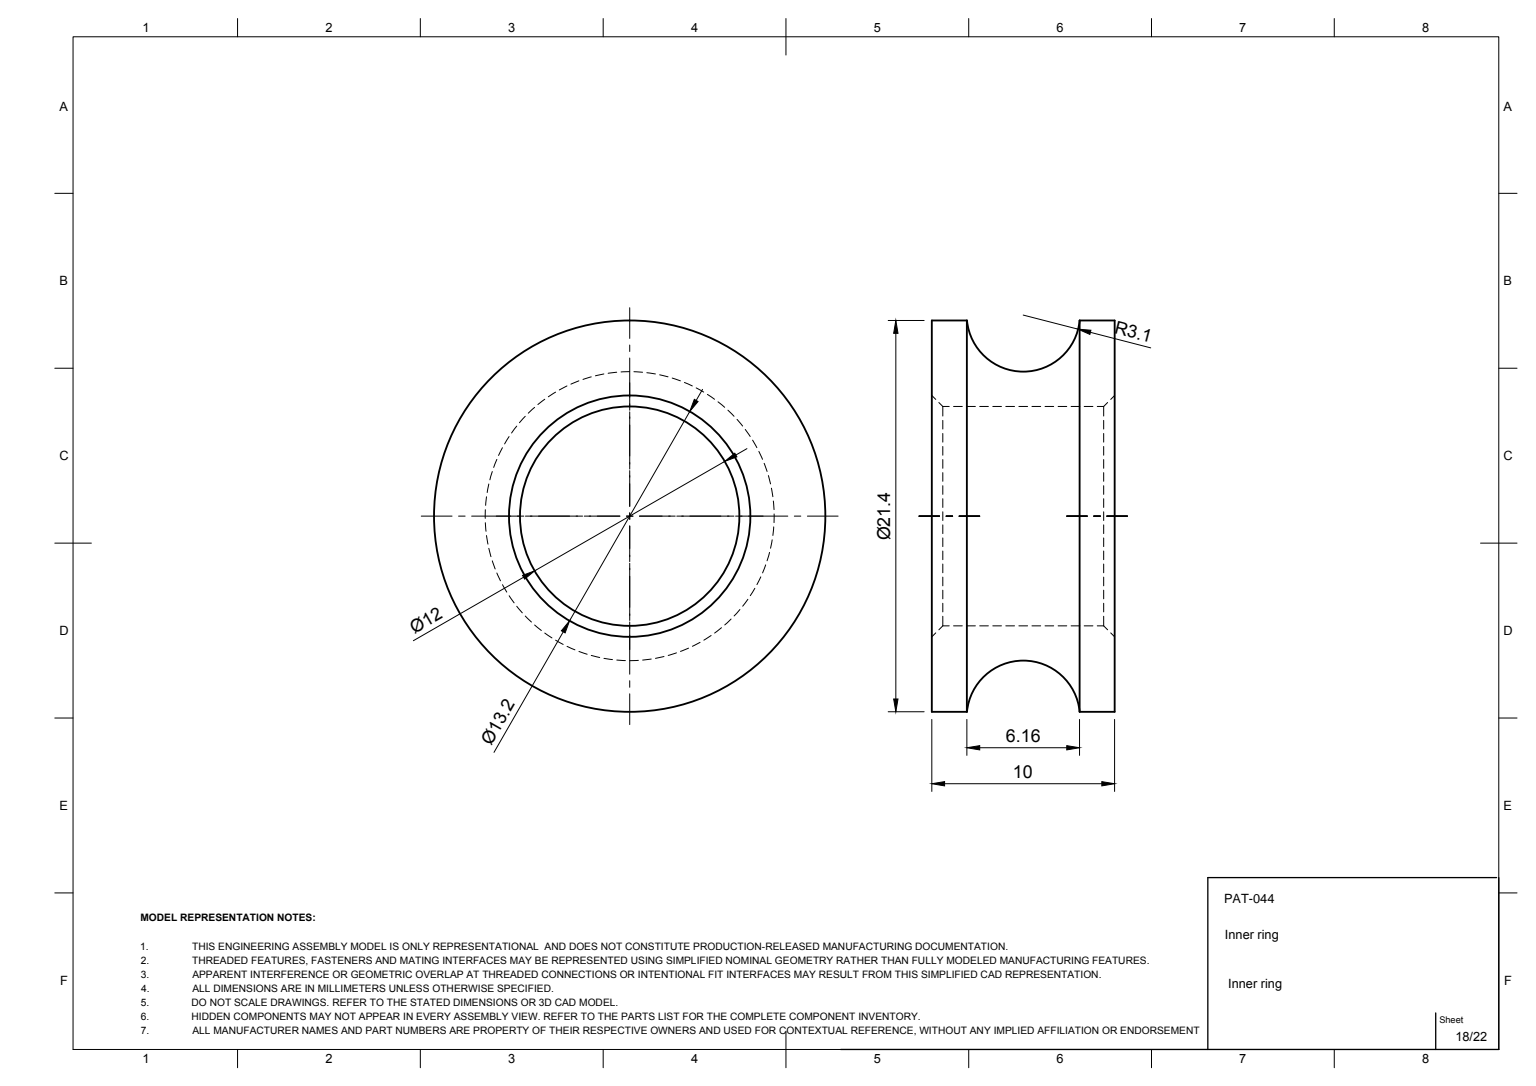
ISO-10303-21;
HEADER;
/* Generated by software containing ST-Developer
 * from STEP Tools, Inc. (www.steptools.com) 
 */

FILE_DESCRIPTION(
/* description */ ('Four-wheel beam trolley'),
/* implementation_level */ '2;1');

FILE_NAME(
/* name */ 'Inner ring.step',
/* time_stamp */ '2026-10-29T16:22:06-07:00',
/* author */ (''),
/* organization */ (''),
/* preprocessor_version */ 'ST-DEVELOPER v20.2',
/* originating_system */ 'Autodesk Translation Framework v15.17.0.0',
/* authorisation */ '');

FILE_SCHEMA (('AUTOMOTIVE_DESIGN { 1 0 10303 214 3 1 1 }'));
ENDSEC;

DATA;
#10=MECHANICAL_DESIGN_GEOMETRIC_PRESENTATION_REPRESENTATION('',(#289),#4777);
#39=TOROIDAL_SURFACE('',#2787,1.1,0.309556);
#238=CONICAL_SURFACE('',#2798,0.63,0.785398163397448);
#239=CONICAL_SURFACE('',#2805,0.63,0.785398163397448);
#255=SHAPE_REPRESENTATION_RELATIONSHIP('SRR','None',#4886,#272);
#272=ADVANCED_BREP_SHAPE_REPRESENTATION('',(#311),#4771);
#289=STYLED_ITEM('',(#5056),#311);
#311=MANIFOLD_SOLID_BREP('Body1',#2378);
#354=FACE_BOUND('',#719,.T.);
#355=FACE_BOUND('',#722,.T.);
#424=PLANE('',#2800);
#425=PLANE('',#2803);
#537=FACE_OUTER_BOUND('',#714,.T.);
#538=FACE_OUTER_BOUND('',#715,.T.);
#539=FACE_OUTER_BOUND('',#716,.T.);
#540=FACE_OUTER_BOUND('',#717,.T.);
#541=FACE_OUTER_BOUND('',#718,.T.);
#542=FACE_OUTER_BOUND('',#720,.T.);
#543=FACE_OUTER_BOUND('',#721,.T.);
#544=FACE_OUTER_BOUND('',#723,.T.);
#714=EDGE_LOOP('',(#1965,#1966,#1967,#1968,#1969,#1970));
#715=EDGE_LOOP('',(#1971,#1972,#1973,#1974,#1975));
#716=EDGE_LOOP('',(#1976,#1977,#1978,#1979));
#717=EDGE_LOOP('',(#1980,#1981,#1982,#1983));
#718=EDGE_LOOP('',(#1984));
#719=EDGE_LOOP('',(#1985));
#720=EDGE_LOOP('',(#1986,#1987,#1988,#1989,#1990));
#721=EDGE_LOOP('',(#1991));
#722=EDGE_LOOP('',(#1992));
#723=EDGE_LOOP('',(#1993,#1994,#1995,#1996));
#882=LINE('',#4197,#1005);
#883=LINE('',#4203,#1006);
#884=LINE('',#4207,#1007);
#885=LINE('',#4213,#1008);
#886=LINE('',#4218,#1009);
#1005=VECTOR('',#3467,1.070235);
#1006=VECTOR('',#3474,0.6);
#1007=VECTOR('',#3479,0.63);
#1008=VECTOR('',#3488,1.070235);
#1009=VECTOR('',#3495,0.63);
#1088=CIRCLE('',#2788,1.070235);
#1089=CIRCLE('',#2789,1.070235);
#1090=CIRCLE('',#2790,0.309556);
#1091=CIRCLE('',#2791,1.070235);
#1092=CIRCLE('',#2792,1.070235);
#1093=CIRCLE('',#2794,1.070235);
#1094=CIRCLE('',#2796,0.6);
#1095=CIRCLE('',#2797,0.6);
#1096=CIRCLE('',#2799,0.66);
#1097=CIRCLE('',#2802,1.070235);
#1098=CIRCLE('',#2804,0.66);
#1272=VERTEX_POINT('',#4186);
#1273=VERTEX_POINT('',#4187);
#1274=VERTEX_POINT('',#4190);
#1275=VERTEX_POINT('',#4192);
#1276=VERTEX_POINT('',#4196);
#1277=VERTEX_POINT('',#4200);
#1278=VERTEX_POINT('',#4202);
#1279=VERTEX_POINT('',#4206);
#1280=VERTEX_POINT('',#4211);
#1281=VERTEX_POINT('',#4215);
#1520=EDGE_CURVE('',#1272,#1273,#1088,.T.);
#1521=EDGE_CURVE('',#1273,#1272,#1089,.T.);
#1522=EDGE_CURVE('',#1273,#1274,#1090,.T.);
#1523=EDGE_CURVE('',#1275,#1274,#1091,.T.);
#1524=EDGE_CURVE('',#1274,#1275,#1092,.T.);
#1525=EDGE_CURVE('',#1275,#1276,#882,.T.);
#1526=EDGE_CURVE('',#1276,#1276,#1093,.T.);
#1527=EDGE_CURVE('',#1277,#1277,#1094,.T.);
#1528=EDGE_CURVE('',#1277,#1278,#883,.T.);
#1529=EDGE_CURVE('',#1278,#1278,#1095,.T.);
#1530=EDGE_CURVE('',#1278,#1279,#884,.T.);
#1531=EDGE_CURVE('',#1279,#1279,#1096,.T.);
#1532=EDGE_CURVE('',#1280,#1280,#1097,.T.);
#1533=EDGE_CURVE('',#1280,#1272,#885,.T.);
#1534=EDGE_CURVE('',#1281,#1281,#1098,.T.);
#1535=EDGE_CURVE('',#1281,#1277,#886,.T.);
#1965=ORIENTED_EDGE('',*,*,#1520,.F.);
#1966=ORIENTED_EDGE('',*,*,#1521,.F.);
#1967=ORIENTED_EDGE('',*,*,#1522,.T.);
#1968=ORIENTED_EDGE('',*,*,#1523,.F.);
#1969=ORIENTED_EDGE('',*,*,#1524,.F.);
#1970=ORIENTED_EDGE('',*,*,#1522,.F.);
#1971=ORIENTED_EDGE('',*,*,#1523,.T.);
#1972=ORIENTED_EDGE('',*,*,#1524,.T.);
#1973=ORIENTED_EDGE('',*,*,#1525,.T.);
#1974=ORIENTED_EDGE('',*,*,#1526,.T.);
#1975=ORIENTED_EDGE('',*,*,#1525,.F.);
#1976=ORIENTED_EDGE('',*,*,#1527,.T.);
#1977=ORIENTED_EDGE('',*,*,#1528,.T.);
#1978=ORIENTED_EDGE('',*,*,#1529,.F.);
#1979=ORIENTED_EDGE('',*,*,#1528,.F.);
#1980=ORIENTED_EDGE('',*,*,#1529,.T.);
#1981=ORIENTED_EDGE('',*,*,#1530,.T.);
#1982=ORIENTED_EDGE('',*,*,#1531,.F.);
#1983=ORIENTED_EDGE('',*,*,#1530,.F.);
#1984=ORIENTED_EDGE('',*,*,#1526,.F.);
#1985=ORIENTED_EDGE('',*,*,#1531,.T.);
#1986=ORIENTED_EDGE('',*,*,#1532,.F.);
#1987=ORIENTED_EDGE('',*,*,#1533,.T.);
#1988=ORIENTED_EDGE('',*,*,#1520,.T.);
#1989=ORIENTED_EDGE('',*,*,#1521,.T.);
#1990=ORIENTED_EDGE('',*,*,#1533,.F.);
#1991=ORIENTED_EDGE('',*,*,#1532,.T.);
#1992=ORIENTED_EDGE('',*,*,#1534,.F.);
#1993=ORIENTED_EDGE('',*,*,#1534,.T.);
#1994=ORIENTED_EDGE('',*,*,#1535,.T.);
#1995=ORIENTED_EDGE('',*,*,#1527,.F.);
#1996=ORIENTED_EDGE('',*,*,#1535,.F.);
#2204=CYLINDRICAL_SURFACE('',#2793,1.070235);
#2205=CYLINDRICAL_SURFACE('',#2795,0.6);
#2206=CYLINDRICAL_SURFACE('',#2801,1.070235);
#2313=ADVANCED_FACE('',(#537),#39,.F.);
#2314=ADVANCED_FACE('',(#538),#2204,.T.);
#2315=ADVANCED_FACE('',(#539),#2205,.F.);
#2316=ADVANCED_FACE('',(#540),#238,.F.);
#2317=ADVANCED_FACE('',(#541,#354),#424,.T.);
#2318=ADVANCED_FACE('',(#542),#2206,.T.);
#2319=ADVANCED_FACE('',(#543,#355),#425,.T.);
#2320=ADVANCED_FACE('',(#544),#239,.F.);
#2378=CLOSED_SHELL('',(#2313,#2314,#2315,#2316,#2317,#2318,#2319,#2320));
#2786=AXIS2_PLACEMENT_3D('',#4184,#3451,#3452);
#2787=AXIS2_PLACEMENT_3D('',#4185,#3453,#3454);
#2788=AXIS2_PLACEMENT_3D('',#4188,#3455,#3456);
#2789=AXIS2_PLACEMENT_3D('',#4189,#3457,#3458);
#2790=AXIS2_PLACEMENT_3D('',#4191,#3459,#3460);
#2791=AXIS2_PLACEMENT_3D('',#4193,#3461,#3462);
#2792=AXIS2_PLACEMENT_3D('',#4194,#3463,#3464);
#2793=AXIS2_PLACEMENT_3D('',#4195,#3465,#3466);
#2794=AXIS2_PLACEMENT_3D('',#4198,#3468,#3469);
#2795=AXIS2_PLACEMENT_3D('',#4199,#3470,#3471);
#2796=AXIS2_PLACEMENT_3D('',#4201,#3472,#3473);
#2797=AXIS2_PLACEMENT_3D('',#4204,#3475,#3476);
#2798=AXIS2_PLACEMENT_3D('',#4205,#3477,#3478);
#2799=AXIS2_PLACEMENT_3D('',#4208,#3480,#3481);
#2800=AXIS2_PLACEMENT_3D('',#4209,#3482,#3483);
#2801=AXIS2_PLACEMENT_3D('',#4210,#3484,#3485);
#2802=AXIS2_PLACEMENT_3D('',#4212,#3486,#3487);
#2803=AXIS2_PLACEMENT_3D('',#4214,#3489,#3490);
#2804=AXIS2_PLACEMENT_3D('',#4216,#3491,#3492);
#2805=AXIS2_PLACEMENT_3D('',#4217,#3493,#3494);
#3451=DIRECTION('axis',(0.,0.,1.));
#3452=DIRECTION('refdir',(1.,0.,0.));
#3453=DIRECTION('center_axis',(0.,-1.,0.));
#3454=DIRECTION('ref_axis',(0.,0.,-1.));
#3455=DIRECTION('center_axis',(0.,-1.,0.));
#3456=DIRECTION('ref_axis',(1.,0.,0.));
#3457=DIRECTION('center_axis',(0.,-1.,0.));
#3458=DIRECTION('ref_axis',(1.,0.,0.));
#3459=DIRECTION('center_axis',(1.,0.,1.22464679914735E-16));
#3460=DIRECTION('ref_axis',(-1.22464679914735E-16,0.,1.));
#3461=DIRECTION('center_axis',(0.,1.,0.));
#3462=DIRECTION('ref_axis',(1.,0.,0.));
#3463=DIRECTION('center_axis',(0.,1.,0.));
#3464=DIRECTION('ref_axis',(1.,0.,0.));
#3465=DIRECTION('center_axis',(0.,-1.,0.));
#3466=DIRECTION('ref_axis',(1.,0.,0.));
#3467=DIRECTION('',(0.,1.,0.));
#3468=DIRECTION('center_axis',(0.,-1.,0.));
#3469=DIRECTION('ref_axis',(1.,0.,0.));
#3470=DIRECTION('center_axis',(0.,-1.,0.));
#3471=DIRECTION('ref_axis',(1.,0.,0.));
#3472=DIRECTION('center_axis',(0.,-1.,0.));
#3473=DIRECTION('ref_axis',(1.,0.,0.));
#3474=DIRECTION('',(0.,1.,0.));
#3475=DIRECTION('center_axis',(0.,-1.,0.));
#3476=DIRECTION('ref_axis',(1.,0.,0.));
#3477=DIRECTION('center_axis',(0.,1.,0.));
#3478=DIRECTION('ref_axis',(1.,0.,0.));
#3479=DIRECTION('',(-0.707106781186548,0.707106781186547,-8.65956056235493E-17));
#3480=DIRECTION('center_axis',(0.,-1.,0.));
#3481=DIRECTION('ref_axis',(1.,0.,0.));
#3482=DIRECTION('center_axis',(0.,1.,0.));
#3483=DIRECTION('ref_axis',(0.,0.,1.));
#3484=DIRECTION('center_axis',(0.,-1.,0.));
#3485=DIRECTION('ref_axis',(1.,0.,0.));
#3486=DIRECTION('center_axis',(0.,-1.,0.));
#3487=DIRECTION('ref_axis',(1.,0.,0.));
#3488=DIRECTION('',(0.,1.,0.));
#3489=DIRECTION('center_axis',(0.,-1.,0.));
#3490=DIRECTION('ref_axis',(0.,0.,-1.));
#3491=DIRECTION('center_axis',(0.,-1.,0.));
#3492=DIRECTION('ref_axis',(1.,0.,0.));
#3493=DIRECTION('center_axis',(0.,-1.,0.));
#3494=DIRECTION('ref_axis',(1.,0.,0.));
#3495=DIRECTION('',(0.707106781186548,0.707106781186547,8.65956056235493E-17));
#4184=CARTESIAN_POINT('',(0.,0.,0.));
#4185=CARTESIAN_POINT('Origin',(0.,0.,0.));
#4186=CARTESIAN_POINT('',(-1.070235,-0.308121667383195,-1.31065986708547E-16));
#4187=CARTESIAN_POINT('',(-1.31065986708547E-16,-0.308121667383195,1.070235));
#4188=CARTESIAN_POINT('Origin',(0.,-0.308121667383195,0.));
#4189=CARTESIAN_POINT('Origin',(0.,-0.308121667383195,0.));
#4190=CARTESIAN_POINT('',(-1.31065986708547E-16,0.308121667383195,1.070235));
#4191=CARTESIAN_POINT('Origin',(-1.34711147906209E-16,0.,1.1));
#4192=CARTESIAN_POINT('',(-1.070235,0.308121667383195,1.31065986708547E-16));
#4193=CARTESIAN_POINT('Origin',(0.,0.308121667383195,0.));
#4194=CARTESIAN_POINT('Origin',(0.,0.308121667383195,0.));
#4195=CARTESIAN_POINT('Origin',(0.,0.,0.));
#4196=CARTESIAN_POINT('',(-1.070235,0.5,-1.31065986708547E-16));
#4197=CARTESIAN_POINT('',(-1.070235,0.,-1.31065986708547E-16));
#4198=CARTESIAN_POINT('Origin',(0.,0.5,0.));
#4199=CARTESIAN_POINT('Origin',(0.,0.,0.));
#4200=CARTESIAN_POINT('',(-0.6,-0.44,-7.34788079488412E-17));
#4201=CARTESIAN_POINT('Origin',(0.,-0.44,0.));
#4202=CARTESIAN_POINT('',(-0.6,0.44,-7.34788079488412E-17));
#4203=CARTESIAN_POINT('',(-0.6,0.,-7.34788079488412E-17));
#4204=CARTESIAN_POINT('Origin',(0.,0.44,0.));
#4205=CARTESIAN_POINT('Origin',(0.,0.47,0.));
#4206=CARTESIAN_POINT('',(-0.66,0.5,-8.08266887437253E-17));
#4207=CARTESIAN_POINT('',(-0.63,0.47,-7.71527483462832E-17));
#4208=CARTESIAN_POINT('Origin',(0.,0.5,0.));
#4209=CARTESIAN_POINT('Origin',(1.070235,0.5,0.));
#4210=CARTESIAN_POINT('Origin',(0.,0.,0.));
#4211=CARTESIAN_POINT('',(-1.070235,-0.5,-1.31065986708547E-16));
#4212=CARTESIAN_POINT('Origin',(0.,-0.5,0.));
#4213=CARTESIAN_POINT('',(-1.070235,0.,-1.31065986708547E-16));
#4214=CARTESIAN_POINT('Origin',(0.66,-0.5,0.));
#4215=CARTESIAN_POINT('',(-0.66,-0.5,-8.08266887437253E-17));
#4216=CARTESIAN_POINT('Origin',(0.,-0.5,0.));
#4217=CARTESIAN_POINT('Origin',(0.,-0.47,0.));
#4218=CARTESIAN_POINT('',(-0.63,-0.47,-7.71527483462832E-17));
#4749=UNCERTAINTY_MEASURE_WITH_UNIT(LENGTH_MEASURE(0.001),#4778,
'DISTANCE_ACCURACY_VALUE',
'Maximum model space distance between geometric entities at asserted c
onnectivities');
#4755=UNCERTAINTY_MEASURE_WITH_UNIT(LENGTH_MEASURE(0.001),#4778,
'DISTANCE_ACCURACY_VALUE',
'Maximum model space distance between geometric entities at asserted c
onnectivities');
#4771=(
GEOMETRIC_REPRESENTATION_CONTEXT(3)
GLOBAL_UNCERTAINTY_ASSIGNED_CONTEXT((#4749))
GLOBAL_UNIT_ASSIGNED_CONTEXT((#4778,#4780,#4781))
REPRESENTATION_CONTEXT('','3D')
);
#4777=(
GEOMETRIC_REPRESENTATION_CONTEXT(3)
GLOBAL_UNCERTAINTY_ASSIGNED_CONTEXT((#4755))
GLOBAL_UNIT_ASSIGNED_CONTEXT((#4778,#4780,#4781))
REPRESENTATION_CONTEXT('','3D')
);
#4778=(
LENGTH_UNIT()
NAMED_UNIT(*)
SI_UNIT(.CENTI.,.METRE.)
);
#4780=(
NAMED_UNIT(*)
PLANE_ANGLE_UNIT()
SI_UNIT($,.RADIAN.)
);
#4781=(
NAMED_UNIT(*)
SI_UNIT($,.STERADIAN.)
SOLID_ANGLE_UNIT()
);
#4797=SHAPE_DEFINITION_REPRESENTATION(#4850,#4886);
#4850=PRODUCT_DEFINITION_SHAPE('',$,#4908);
#4886=SHAPE_REPRESENTATION('',(#2786),#4771);
#4892=PRODUCT_DEFINITION_CONTEXT('part definition',#4957,'design');
#4908=PRODUCT_DEFINITION('Inner ring','Inner ring',#4929,#4892);
#4929=PRODUCT_DEFINITION_FORMATION('',$,#4974);
#4957=APPLICATION_CONTEXT(
'Core Data for Automotive Mechanical Design Process');
#4958=PRODUCT_CONTEXT('part definition',#4957,'mechanical');
#4974=PRODUCT('Inner ring','Inner ring','Inner ring',(#4958));
#5050=COLOUR_RGB('Grey',0.48,0.52,0.57);
#5051=FILL_AREA_STYLE_COLOUR('',#5050);
#5052=FILL_AREA_STYLE('',(#5051));
#5053=SURFACE_STYLE_FILL_AREA(#5052);
#5054=SURFACE_SIDE_STYLE('',(#5053));
#5055=SURFACE_STYLE_USAGE(.BOTH.,#5054);
#5056=PRESENTATION_STYLE_ASSIGNMENT((#5055));
ENDSEC;
END-ISO-10303-21;
